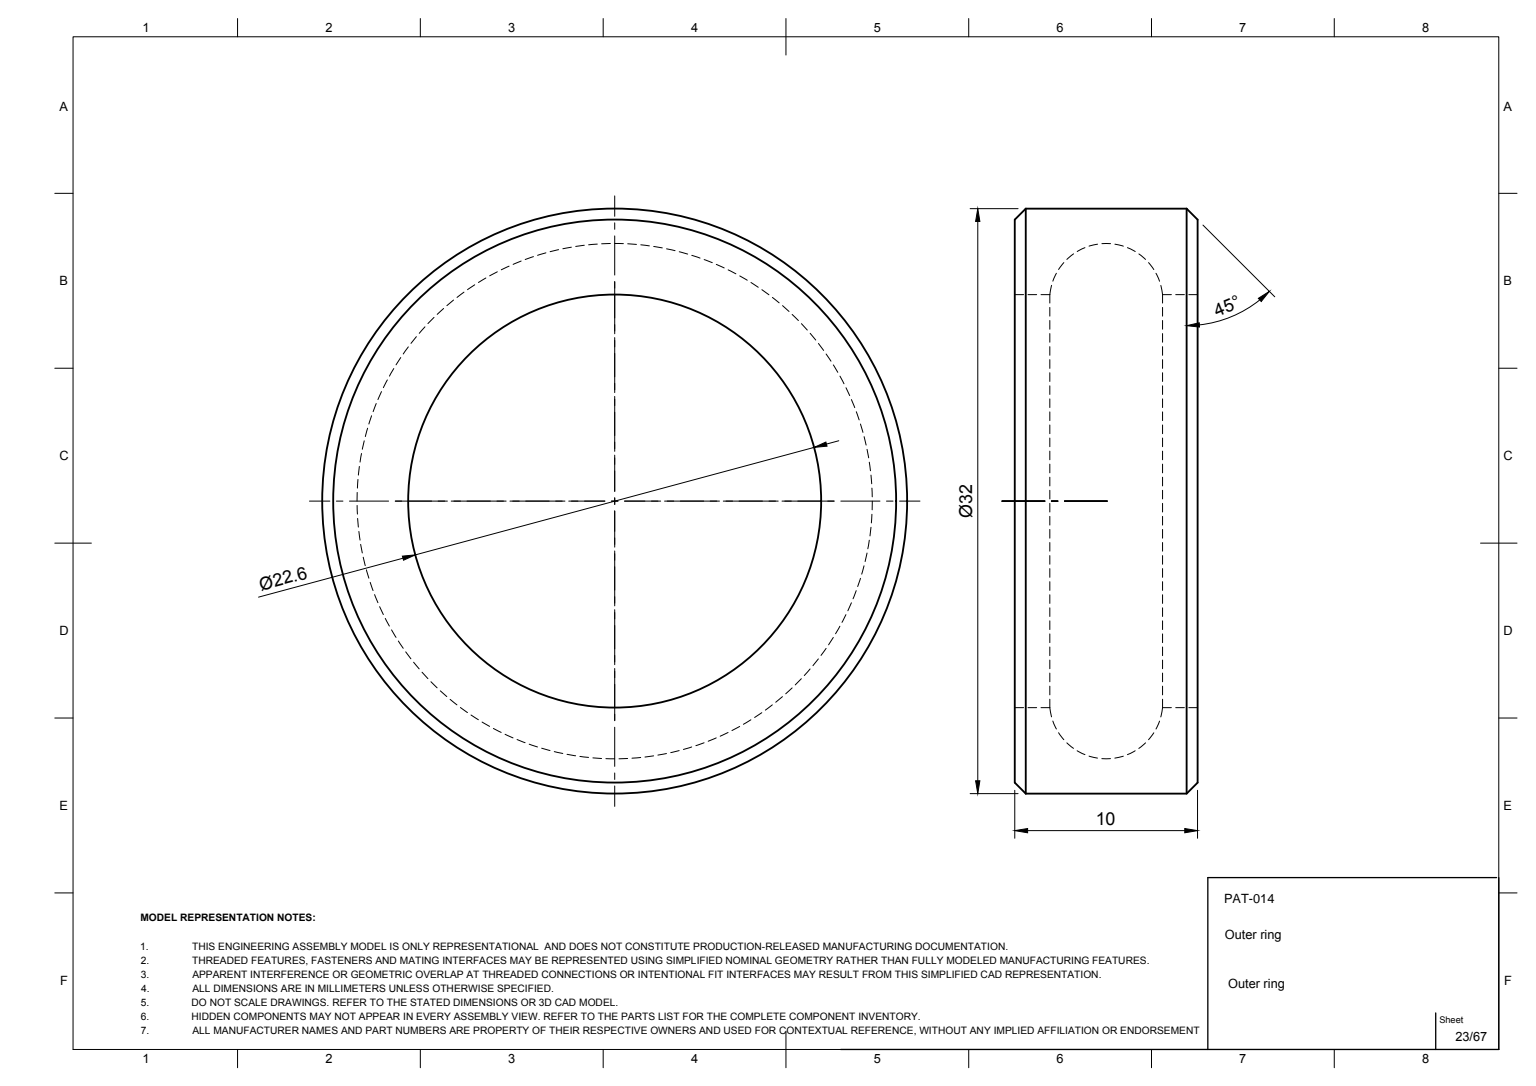
ISO-10303-21;
HEADER;
/* Generated by software containing ST-Developer
 * from STEP Tools, Inc. (www.steptools.com) 
 */

FILE_DESCRIPTION(
/* description */ ('Bin tilter linkage'),
/* implementation_level */ '2;1');

FILE_NAME(
/* name */ 'Outer ring.step',
/* time_stamp */ '2026-10-28T03:26:24-07:00',
/* author */ (''),
/* organization */ (''),
/* preprocessor_version */ 'ST-DEVELOPER v20.2',
/* originating_system */ 'Autodesk Translation Framework v15.17.0.0',
/* authorisation */ '');

FILE_SCHEMA (('AUTOMOTIVE_DESIGN { 1 0 10303 214 3 1 1 }'));
ENDSEC;

DATA;
#10=MECHANICAL_DESIGN_GEOMETRIC_PRESENTATION_REPRESENTATION('',(#935),#23728);
#628=TOROIDAL_SURFACE('',#14795,1.1,0.309556);
#638=CONICAL_SURFACE('',#14806,1.57,0.785398163397449);
#639=CONICAL_SURFACE('',#14810,1.57,0.785398163397449);
#723=SHAPE_REPRESENTATION_RELATIONSHIP('SRR','None',#24190,#829);
#829=ADVANCED_BREP_SHAPE_REPRESENTATION('',(#1048),#23690);
#935=STYLED_ITEM('',(#24765),#1048);
#1048=MANIFOLD_SOLID_BREP('Body1',#12466);
#1388=FACE_BOUND('',#3484,.T.);
#1389=FACE_BOUND('',#3489,.T.);
#1739=PLANE('',#14803);
#1740=PLANE('',#14812);
#2403=FACE_OUTER_BOUND('',#3481,.T.);
#2404=FACE_OUTER_BOUND('',#3482,.T.);
#2405=FACE_OUTER_BOUND('',#3483,.T.);
#2406=FACE_OUTER_BOUND('',#3485,.T.);
#2407=FACE_OUTER_BOUND('',#3486,.T.);
#2408=FACE_OUTER_BOUND('',#3487,.T.);
#2409=FACE_OUTER_BOUND('',#3488,.T.);
#2410=FACE_OUTER_BOUND('',#3490,.T.);
#3481=EDGE_LOOP('',(#10245,#10246,#10247,#10248,#10249,#10250));
#3482=EDGE_LOOP('',(#10251,#10252,#10253,#10254,#10255));
#3483=EDGE_LOOP('',(#10256));
#3484=EDGE_LOOP('',(#10257));
#3485=EDGE_LOOP('',(#10258,#10259,#10260,#10261));
#3486=EDGE_LOOP('',(#10262,#10263,#10264,#10265));
#3487=EDGE_LOOP('',(#10266,#10267,#10268,#10269));
#3488=EDGE_LOOP('',(#10270));
#3489=EDGE_LOOP('',(#10271));
#3490=EDGE_LOOP('',(#10272,#10273,#10274,#10275,#10276));
#4258=LINE('',#21908,#4933);
#4259=LINE('',#21917,#4934);
#4260=LINE('',#21921,#4935);
#4261=LINE('',#21925,#4936);
#4262=LINE('',#21928,#4937);
#4933=VECTOR('',#18137,1.129765);
#4934=VECTOR('',#18148,1.57);
#4935=VECTOR('',#18153,1.6);
#4936=VECTOR('',#18158,1.57);
#4937=VECTOR('',#18163,1.129765);
#5726=CIRCLE('',#14796,1.129765);
#5727=CIRCLE('',#14797,1.129765);
#5728=CIRCLE('',#14798,0.309556);
#5729=CIRCLE('',#14799,1.129765);
#5730=CIRCLE('',#14800,1.129765);
#5731=CIRCLE('',#14802,1.129765);
#5732=CIRCLE('',#14804,1.54);
#5733=CIRCLE('',#14805,1.129765);
#5734=CIRCLE('',#14807,1.6);
#5735=CIRCLE('',#14809,1.6);
#5736=CIRCLE('',#14811,1.54);
#6579=VERTEX_POINT('',#21896);
#6580=VERTEX_POINT('',#21897);
#6581=VERTEX_POINT('',#21900);
#6582=VERTEX_POINT('',#21902);
#6583=VERTEX_POINT('',#21906);
#6584=VERTEX_POINT('',#21910);
#6585=VERTEX_POINT('',#21912);
#6586=VERTEX_POINT('',#21915);
#6587=VERTEX_POINT('',#21919);
#6588=VERTEX_POINT('',#21923);
#7862=EDGE_CURVE('',#6579,#6580,#5726,.T.);
#7863=EDGE_CURVE('',#6580,#6579,#5727,.T.);
#7864=EDGE_CURVE('',#6580,#6581,#5728,.T.);
#7865=EDGE_CURVE('',#6582,#6581,#5729,.T.);
#7866=EDGE_CURVE('',#6581,#6582,#5730,.T.);
#7867=EDGE_CURVE('',#6583,#6583,#5731,.T.);
#7868=EDGE_CURVE('',#6583,#6582,#4258,.T.);
#7869=EDGE_CURVE('',#6584,#6584,#5732,.T.);
#7870=EDGE_CURVE('',#6585,#6585,#5733,.T.);
#7871=EDGE_CURVE('',#6586,#6586,#5734,.T.);
#7872=EDGE_CURVE('',#6586,#6584,#4259,.T.);
#7873=EDGE_CURVE('',#6587,#6587,#5735,.T.);
#7874=EDGE_CURVE('',#6587,#6586,#4260,.T.);
#7875=EDGE_CURVE('',#6588,#6588,#5736,.T.);
#7876=EDGE_CURVE('',#6588,#6587,#4261,.T.);
#7877=EDGE_CURVE('',#6579,#6585,#4262,.T.);
#10245=ORIENTED_EDGE('',*,*,#7862,.F.);
#10246=ORIENTED_EDGE('',*,*,#7863,.F.);
#10247=ORIENTED_EDGE('',*,*,#7864,.T.);
#10248=ORIENTED_EDGE('',*,*,#7865,.F.);
#10249=ORIENTED_EDGE('',*,*,#7866,.F.);
#10250=ORIENTED_EDGE('',*,*,#7864,.F.);
#10251=ORIENTED_EDGE('',*,*,#7867,.T.);
#10252=ORIENTED_EDGE('',*,*,#7868,.T.);
#10253=ORIENTED_EDGE('',*,*,#7865,.T.);
#10254=ORIENTED_EDGE('',*,*,#7866,.T.);
#10255=ORIENTED_EDGE('',*,*,#7868,.F.);
#10256=ORIENTED_EDGE('',*,*,#7869,.F.);
#10257=ORIENTED_EDGE('',*,*,#7870,.T.);
#10258=ORIENTED_EDGE('',*,*,#7871,.F.);
#10259=ORIENTED_EDGE('',*,*,#7872,.T.);
#10260=ORIENTED_EDGE('',*,*,#7869,.T.);
#10261=ORIENTED_EDGE('',*,*,#7872,.F.);
#10262=ORIENTED_EDGE('',*,*,#7873,.F.);
#10263=ORIENTED_EDGE('',*,*,#7874,.T.);
#10264=ORIENTED_EDGE('',*,*,#7871,.T.);
#10265=ORIENTED_EDGE('',*,*,#7874,.F.);
#10266=ORIENTED_EDGE('',*,*,#7875,.F.);
#10267=ORIENTED_EDGE('',*,*,#7876,.T.);
#10268=ORIENTED_EDGE('',*,*,#7873,.T.);
#10269=ORIENTED_EDGE('',*,*,#7876,.F.);
#10270=ORIENTED_EDGE('',*,*,#7875,.T.);
#10271=ORIENTED_EDGE('',*,*,#7867,.F.);
#10272=ORIENTED_EDGE('',*,*,#7862,.T.);
#10273=ORIENTED_EDGE('',*,*,#7863,.T.);
#10274=ORIENTED_EDGE('',*,*,#7877,.T.);
#10275=ORIENTED_EDGE('',*,*,#7870,.F.);
#10276=ORIENTED_EDGE('',*,*,#7877,.F.);
#11526=CYLINDRICAL_SURFACE('',#14801,1.129765);
#11527=CYLINDRICAL_SURFACE('',#14808,1.6);
#11528=CYLINDRICAL_SURFACE('',#14813,1.129765);
#12128=ADVANCED_FACE('',(#2403),#628,.F.);
#12129=ADVANCED_FACE('',(#2404),#11526,.F.);
#12130=ADVANCED_FACE('',(#2405,#1388),#1739,.T.);
#12131=ADVANCED_FACE('',(#2406),#638,.T.);
#12132=ADVANCED_FACE('',(#2407),#11527,.T.);
#12133=ADVANCED_FACE('',(#2408),#639,.T.);
#12134=ADVANCED_FACE('',(#2409,#1389),#1740,.T.);
#12135=ADVANCED_FACE('',(#2410),#11528,.F.);
#12466=CLOSED_SHELL('',(#12128,#12129,#12130,#12131,#12132,#12133,#12134,
#12135));
#14794=AXIS2_PLACEMENT_3D('',#21894,#18119,#18120);
#14795=AXIS2_PLACEMENT_3D('',#21895,#18121,#18122);
#14796=AXIS2_PLACEMENT_3D('',#21898,#18123,#18124);
#14797=AXIS2_PLACEMENT_3D('',#21899,#18125,#18126);
#14798=AXIS2_PLACEMENT_3D('',#21901,#18127,#18128);
#14799=AXIS2_PLACEMENT_3D('',#21903,#18129,#18130);
#14800=AXIS2_PLACEMENT_3D('',#21904,#18131,#18132);
#14801=AXIS2_PLACEMENT_3D('',#21905,#18133,#18134);
#14802=AXIS2_PLACEMENT_3D('',#21907,#18135,#18136);
#14803=AXIS2_PLACEMENT_3D('',#21909,#18138,#18139);
#14804=AXIS2_PLACEMENT_3D('',#21911,#18140,#18141);
#14805=AXIS2_PLACEMENT_3D('',#21913,#18142,#18143);
#14806=AXIS2_PLACEMENT_3D('',#21914,#18144,#18145);
#14807=AXIS2_PLACEMENT_3D('',#21916,#18146,#18147);
#14808=AXIS2_PLACEMENT_3D('',#21918,#18149,#18150);
#14809=AXIS2_PLACEMENT_3D('',#21920,#18151,#18152);
#14810=AXIS2_PLACEMENT_3D('',#21922,#18154,#18155);
#14811=AXIS2_PLACEMENT_3D('',#21924,#18156,#18157);
#14812=AXIS2_PLACEMENT_3D('',#21926,#18159,#18160);
#14813=AXIS2_PLACEMENT_3D('',#21927,#18161,#18162);
#18119=DIRECTION('axis',(0.,0.,1.));
#18120=DIRECTION('refdir',(1.,0.,0.));
#18121=DIRECTION('center_axis',(0.,-1.,0.));
#18122=DIRECTION('ref_axis',(0.,0.,-1.));
#18123=DIRECTION('center_axis',(0.,-1.,0.));
#18124=DIRECTION('ref_axis',(1.,0.,0.));
#18125=DIRECTION('center_axis',(0.,-1.,0.));
#18126=DIRECTION('ref_axis',(1.,0.,0.));
#18127=DIRECTION('center_axis',(1.,0.,1.22464679914735E-16));
#18128=DIRECTION('ref_axis',(-1.22464679914735E-16,0.,1.));
#18129=DIRECTION('center_axis',(0.,1.,0.));
#18130=DIRECTION('ref_axis',(1.,0.,0.));
#18131=DIRECTION('center_axis',(0.,1.,0.));
#18132=DIRECTION('ref_axis',(1.,0.,0.));
#18133=DIRECTION('center_axis',(0.,-1.,0.));
#18134=DIRECTION('ref_axis',(1.,0.,0.));
#18135=DIRECTION('center_axis',(0.,-1.,0.));
#18136=DIRECTION('ref_axis',(1.,0.,0.));
#18137=DIRECTION('',(0.,1.,0.));
#18138=DIRECTION('center_axis',(0.,1.,0.));
#18139=DIRECTION('ref_axis',(0.,0.,1.));
#18140=DIRECTION('center_axis',(0.,-1.,0.));
#18141=DIRECTION('ref_axis',(1.,0.,0.));
#18142=DIRECTION('center_axis',(0.,-1.,0.));
#18143=DIRECTION('ref_axis',(1.,0.,0.));
#18144=DIRECTION('center_axis',(0.,-1.,0.));
#18145=DIRECTION('ref_axis',(1.,0.,0.));
#18146=DIRECTION('center_axis',(0.,-1.,0.));
#18147=DIRECTION('ref_axis',(1.,0.,0.));
#18148=DIRECTION('',(0.707106781186548,0.707106781186547,8.65956056235494E-17));
#18149=DIRECTION('center_axis',(0.,-1.,0.));
#18150=DIRECTION('ref_axis',(1.,0.,0.));
#18151=DIRECTION('center_axis',(0.,-1.,0.));
#18152=DIRECTION('ref_axis',(1.,0.,0.));
#18153=DIRECTION('',(0.,1.,0.));
#18154=DIRECTION('center_axis',(0.,1.,0.));
#18155=DIRECTION('ref_axis',(1.,0.,0.));
#18156=DIRECTION('center_axis',(0.,-1.,0.));
#18157=DIRECTION('ref_axis',(1.,0.,0.));
#18158=DIRECTION('',(-0.707106781186548,0.707106781186547,-8.65956056235494E-17));
#18159=DIRECTION('center_axis',(0.,-1.,0.));
#18160=DIRECTION('ref_axis',(0.,0.,-1.));
#18161=DIRECTION('center_axis',(0.,-1.,0.));
#18162=DIRECTION('ref_axis',(1.,0.,0.));
#18163=DIRECTION('',(0.,1.,0.));
#21894=CARTESIAN_POINT('',(0.,0.,0.));
#21895=CARTESIAN_POINT('Origin',(0.,0.,0.));
#21896=CARTESIAN_POINT('',(-1.129765,0.308121667383195,-1.38356309103871E-16));
#21897=CARTESIAN_POINT('',(-1.38356309103871E-16,0.308121667383195,1.129765));
#21898=CARTESIAN_POINT('Origin',(0.,0.308121667383195,0.));
#21899=CARTESIAN_POINT('Origin',(0.,0.308121667383195,0.));
#21900=CARTESIAN_POINT('',(-1.38356309103871E-16,-0.308121667383195,1.129765));
#21901=CARTESIAN_POINT('Origin',(-1.34711147906209E-16,0.,1.1));
#21902=CARTESIAN_POINT('',(-1.129765,-0.308121667383195,1.38356309103871E-16));
#21903=CARTESIAN_POINT('Origin',(0.,-0.308121667383195,0.));
#21904=CARTESIAN_POINT('Origin',(0.,-0.308121667383195,0.));
#21905=CARTESIAN_POINT('Origin',(0.,0.,0.));
#21906=CARTESIAN_POINT('',(-1.129765,-0.5,-1.38356309103871E-16));
#21907=CARTESIAN_POINT('Origin',(0.,-0.5,0.));
#21908=CARTESIAN_POINT('',(-1.129765,0.,-1.38356309103871E-16));
#21909=CARTESIAN_POINT('Origin',(1.54,0.5,0.));
#21910=CARTESIAN_POINT('',(-1.54,0.5,-1.88595607068692E-16));
#21911=CARTESIAN_POINT('Origin',(0.,0.5,0.));
#21912=CARTESIAN_POINT('',(-1.129765,0.5,-1.38356309103871E-16));
#21913=CARTESIAN_POINT('Origin',(0.,0.5,0.));
#21914=CARTESIAN_POINT('Origin',(0.,0.47,0.));
#21915=CARTESIAN_POINT('',(-1.6,0.44,-1.95943487863577E-16));
#21916=CARTESIAN_POINT('Origin',(0.,0.44,0.));
#21917=CARTESIAN_POINT('',(-1.57,0.47,-1.92269547466134E-16));
#21918=CARTESIAN_POINT('Origin',(0.,0.,0.));
#21919=CARTESIAN_POINT('',(-1.6,-0.44,-1.95943487863577E-16));
#21920=CARTESIAN_POINT('Origin',(0.,-0.44,0.));
#21921=CARTESIAN_POINT('',(-1.6,0.,-1.95943487863577E-16));
#21922=CARTESIAN_POINT('Origin',(0.,-0.47,0.));
#21923=CARTESIAN_POINT('',(-1.54,-0.5,-1.88595607068692E-16));
#21924=CARTESIAN_POINT('Origin',(0.,-0.5,0.));
#21925=CARTESIAN_POINT('',(-1.57,-0.47,-1.92269547466134E-16));
#21926=CARTESIAN_POINT('Origin',(1.129765,-0.5,0.));
#21927=CARTESIAN_POINT('Origin',(0.,0.,0.));
#21928=CARTESIAN_POINT('',(-1.129765,0.,-1.38356309103871E-16));
#23573=UNCERTAINTY_MEASURE_WITH_UNIT(LENGTH_MEASURE(0.001),#23729,
'DISTANCE_ACCURACY_VALUE',
'Maximum model space distance between geometric entities at asserted c
onnectivities');
#23611=UNCERTAINTY_MEASURE_WITH_UNIT(LENGTH_MEASURE(0.001),#23729,
'DISTANCE_ACCURACY_VALUE',
'Maximum model space distance between geometric entities at asserted c
onnectivities');
#23690=(
GEOMETRIC_REPRESENTATION_CONTEXT(3)
GLOBAL_UNCERTAINTY_ASSIGNED_CONTEXT((#23573))
GLOBAL_UNIT_ASSIGNED_CONTEXT((#23729,#23731,#23732))
REPRESENTATION_CONTEXT('','3D')
);
#23728=(
GEOMETRIC_REPRESENTATION_CONTEXT(3)
GLOBAL_UNCERTAINTY_ASSIGNED_CONTEXT((#23611))
GLOBAL_UNIT_ASSIGNED_CONTEXT((#23729,#23731,#23732))
REPRESENTATION_CONTEXT('','3D')
);
#23729=(
LENGTH_UNIT()
NAMED_UNIT(*)
SI_UNIT(.CENTI.,.METRE.)
);
#23731=(
NAMED_UNIT(*)
PLANE_ANGLE_UNIT()
SI_UNIT($,.RADIAN.)
);
#23732=(
NAMED_UNIT(*)
SI_UNIT($,.STERADIAN.)
SOLID_ANGLE_UNIT()
);
#23811=SHAPE_DEFINITION_REPRESENTATION(#23927,#24190);
#23927=PRODUCT_DEFINITION_SHAPE('',$,#24307);
#24190=SHAPE_REPRESENTATION('',(#14794),#23690);
#24228=PRODUCT_DEFINITION_CONTEXT('part definition',#24578,'design');
#24307=PRODUCT_DEFINITION('Outer ring','Outer ring',#24423,#24228);
#24423=PRODUCT_DEFINITION_FORMATION('',$,#24658);
#24578=APPLICATION_CONTEXT(
'Core Data for Automotive Mechanical Design Process');
#24579=PRODUCT_CONTEXT('part definition',#24578,'mechanical');
#24658=PRODUCT('Outer ring','Outer ring','Outer ring',(#24579));
#24759=COLOUR_RGB('Grey',0.48,0.52,0.57);
#24760=FILL_AREA_STYLE_COLOUR('',#24759);
#24761=FILL_AREA_STYLE('',(#24760));
#24762=SURFACE_STYLE_FILL_AREA(#24761);
#24763=SURFACE_SIDE_STYLE('',(#24762));
#24764=SURFACE_STYLE_USAGE(.BOTH.,#24763);
#24765=PRESENTATION_STYLE_ASSIGNMENT((#24764));
ENDSEC;
END-ISO-10303-21;
